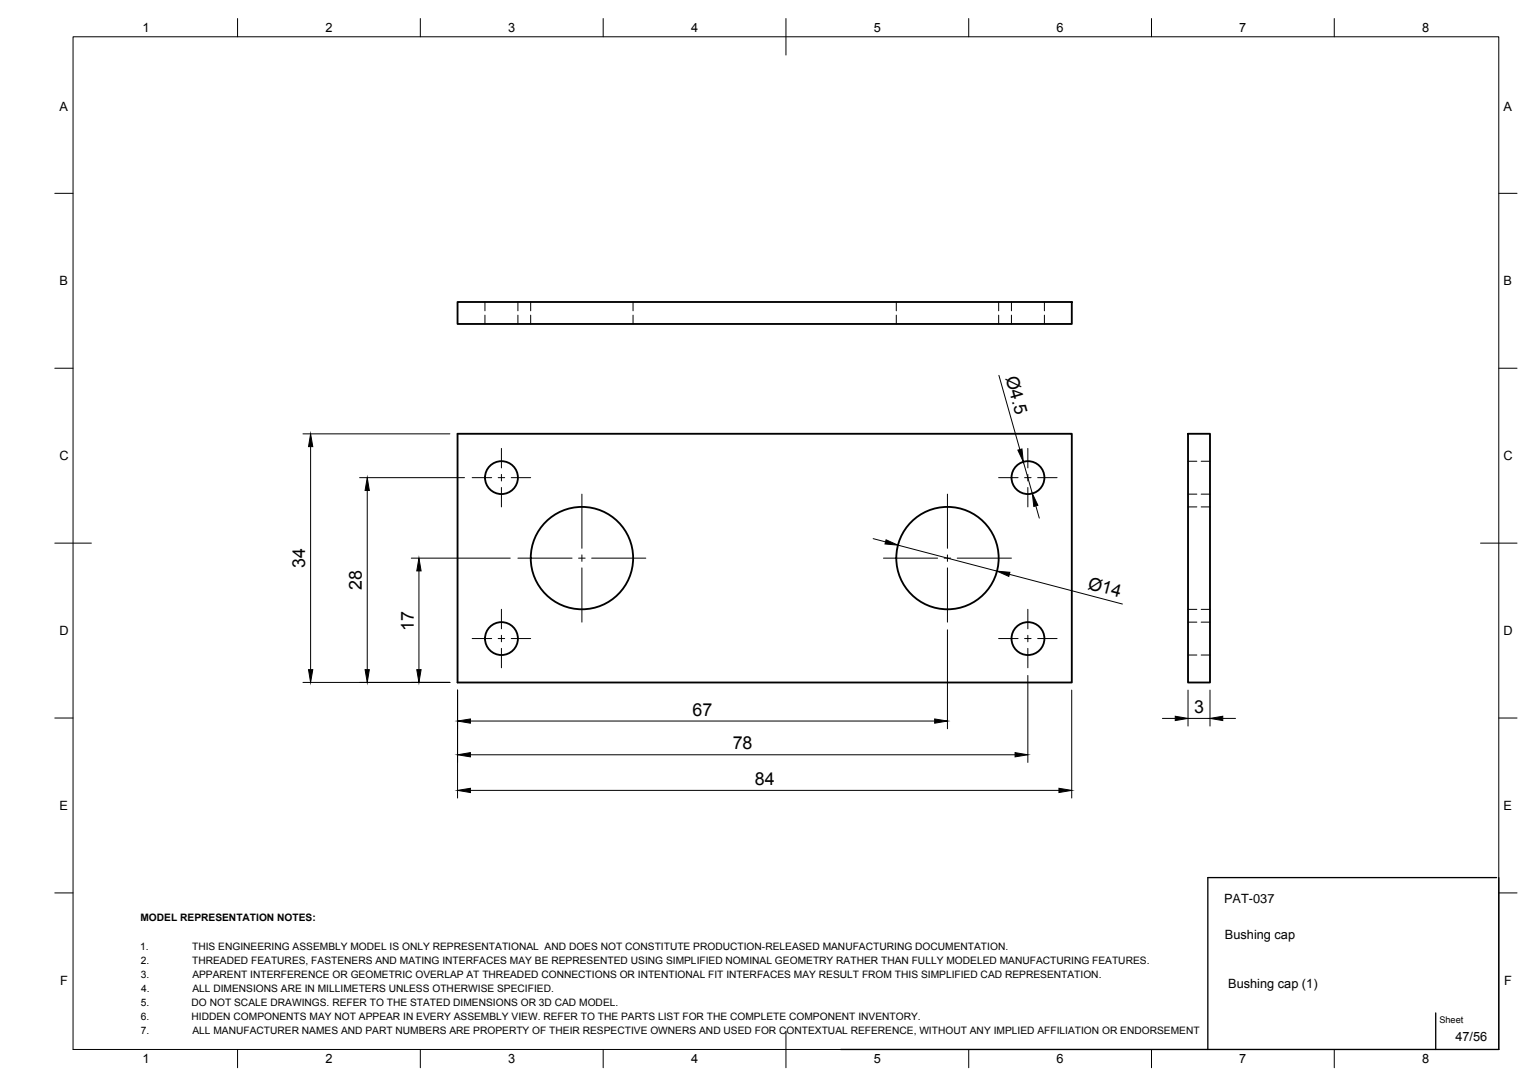
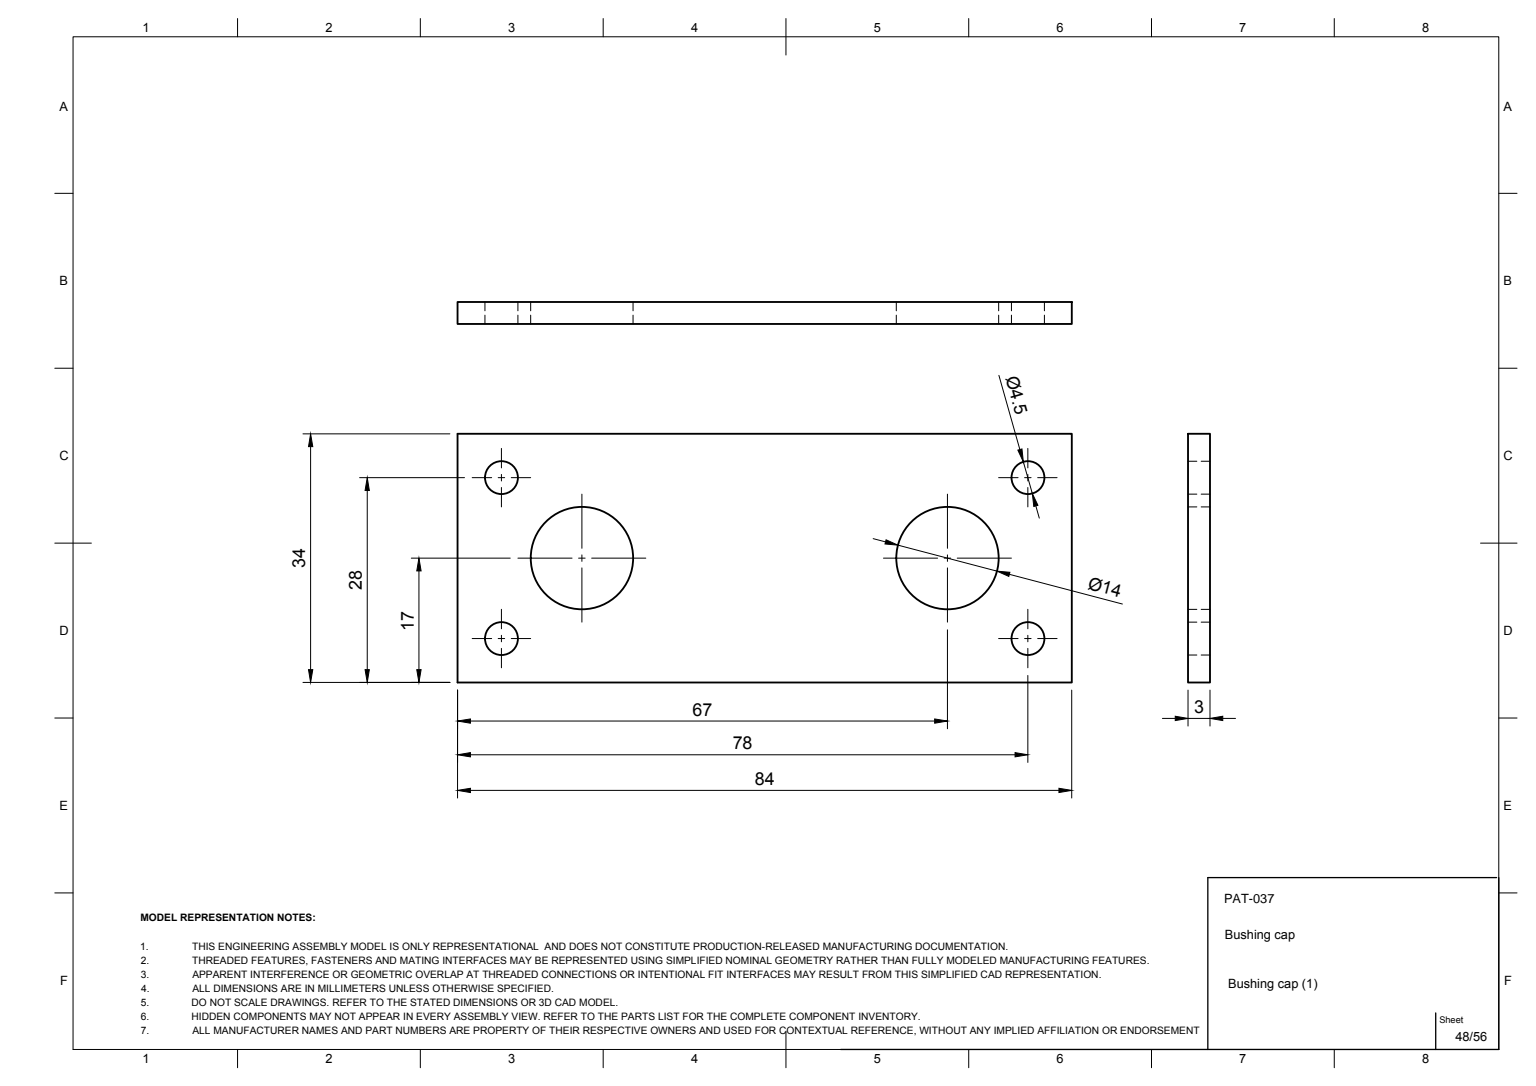
ISO-10303-21;
HEADER;
/* Generated by software containing ST-Developer
 * from STEP Tools, Inc. (www.steptools.com) 
 */

FILE_DESCRIPTION(
/* description */ ('Flywheel Crank-Slider'),
/* implementation_level */ '2;1');

FILE_NAME(
/* name */ 'Bushing cap (1).step',
/* time_stamp */ '2026-10-28T03:23:13-07:00',
/* author */ (''),
/* organization */ (''),
/* preprocessor_version */ 'ST-DEVELOPER v20.2',
/* originating_system */ 'Autodesk Translation Framework v15.17.0.0',
/* authorisation */ '');

FILE_SCHEMA (('AUTOMOTIVE_DESIGN { 1 0 10303 214 3 1 1 }'));
ENDSEC;

DATA;
#10=MECHANICAL_DESIGN_GEOMETRIC_PRESENTATION_REPRESENTATION('',(#721),#17322);
#608=SHAPE_REPRESENTATION_RELATIONSHIP('SRR','None',#17609,#660);
#660=ADVANCED_BREP_SHAPE_REPRESENTATION('',(#778),#17313);
#721=STYLED_ITEM('',(#17924),#778);
#778=MANIFOLD_SOLID_BREP('Body1',#9103);
#979=FACE_BOUND('',#2520,.T.);
#980=FACE_BOUND('',#2521,.T.);
#981=FACE_BOUND('',#2522,.T.);
#982=FACE_BOUND('',#2523,.T.);
#983=FACE_BOUND('',#2524,.T.);
#984=FACE_BOUND('',#2525,.T.);
#985=FACE_BOUND('',#2528,.T.);
#986=FACE_BOUND('',#2529,.T.);
#987=FACE_BOUND('',#2530,.T.);
#988=FACE_BOUND('',#2531,.T.);
#989=FACE_BOUND('',#2532,.T.);
#990=FACE_BOUND('',#2533,.T.);
#1276=PLANE('',#10612);
#1277=PLANE('',#10613);
#1278=PLANE('',#10614);
#1279=PLANE('',#10615);
#1280=PLANE('',#10616);
#1281=PLANE('',#10617);
#1783=FACE_OUTER_BOUND('',#2512,.T.);
#1784=FACE_OUTER_BOUND('',#2513,.T.);
#1785=FACE_OUTER_BOUND('',#2514,.T.);
#1786=FACE_OUTER_BOUND('',#2515,.T.);
#1787=FACE_OUTER_BOUND('',#2516,.T.);
#1788=FACE_OUTER_BOUND('',#2517,.T.);
#1789=FACE_OUTER_BOUND('',#2518,.T.);
#1790=FACE_OUTER_BOUND('',#2519,.T.);
#1791=FACE_OUTER_BOUND('',#2526,.T.);
#1792=FACE_OUTER_BOUND('',#2527,.T.);
#1793=FACE_OUTER_BOUND('',#2534,.T.);
#1794=FACE_OUTER_BOUND('',#2535,.T.);
#2512=EDGE_LOOP('',(#8060,#8061,#8062,#8063));
#2513=EDGE_LOOP('',(#8064,#8065,#8066,#8067));
#2514=EDGE_LOOP('',(#8068,#8069,#8070,#8071));
#2515=EDGE_LOOP('',(#8072,#8073,#8074,#8075));
#2516=EDGE_LOOP('',(#8076,#8077,#8078,#8079));
#2517=EDGE_LOOP('',(#8080,#8081,#8082,#8083));
#2518=EDGE_LOOP('',(#8084,#8085,#8086,#8087));
#2519=EDGE_LOOP('',(#8088,#8089,#8090,#8091));
#2520=EDGE_LOOP('',(#8092));
#2521=EDGE_LOOP('',(#8093));
#2522=EDGE_LOOP('',(#8094));
#2523=EDGE_LOOP('',(#8095));
#2524=EDGE_LOOP('',(#8096));
#2525=EDGE_LOOP('',(#8097));
#2526=EDGE_LOOP('',(#8098,#8099,#8100,#8101));
#2527=EDGE_LOOP('',(#8102,#8103,#8104,#8105));
#2528=EDGE_LOOP('',(#8106));
#2529=EDGE_LOOP('',(#8107));
#2530=EDGE_LOOP('',(#8108));
#2531=EDGE_LOOP('',(#8109));
#2532=EDGE_LOOP('',(#8110));
#2533=EDGE_LOOP('',(#8111));
#2534=EDGE_LOOP('',(#8112,#8113,#8114,#8115));
#2535=EDGE_LOOP('',(#8116,#8117,#8118,#8119));
#3151=LINE('',#16804,#3762);
#3152=LINE('',#16810,#3763);
#3153=LINE('',#16816,#3764);
#3154=LINE('',#16822,#3765);
#3155=LINE('',#16828,#3766);
#3156=LINE('',#16834,#3767);
#3157=LINE('',#16839,#3768);
#3158=LINE('',#16841,#3769);
#3159=LINE('',#16843,#3770);
#3160=LINE('',#16844,#3771);
#3161=LINE('',#16847,#3772);
#3162=LINE('',#16849,#3773);
#3163=LINE('',#16850,#3774);
#3164=LINE('',#16853,#3775);
#3165=LINE('',#16855,#3776);
#3166=LINE('',#16856,#3777);
#3167=LINE('',#16858,#3778);
#3168=LINE('',#16859,#3779);
#3762=VECTOR('',#13187,0.225);
#3763=VECTOR('',#13194,0.225);
#3764=VECTOR('',#13201,0.225);
#3765=VECTOR('',#13208,0.225);
#3766=VECTOR('',#13215,0.7);
#3767=VECTOR('',#13222,0.7);
#3768=VECTOR('',#13227,1.);
#3769=VECTOR('',#13228,1.);
#3770=VECTOR('',#13229,1.);
#3771=VECTOR('',#13230,1.);
#3772=VECTOR('',#13233,1.);
#3773=VECTOR('',#13234,1.);
#3774=VECTOR('',#13235,1.);
#3775=VECTOR('',#13238,1.);
#3776=VECTOR('',#13239,1.);
#3777=VECTOR('',#13240,1.);
#3778=VECTOR('',#13243,1.);
#3779=VECTOR('',#13244,1.);
#4218=CIRCLE('',#10595,0.225);
#4219=CIRCLE('',#10596,0.225);
#4220=CIRCLE('',#10598,0.225);
#4221=CIRCLE('',#10599,0.225);
#4222=CIRCLE('',#10601,0.225);
#4223=CIRCLE('',#10602,0.225);
#4224=CIRCLE('',#10604,0.225);
#4225=CIRCLE('',#10605,0.225);
#4226=CIRCLE('',#10607,0.7);
#4227=CIRCLE('',#10608,0.7);
#4228=CIRCLE('',#10610,0.7);
#4229=CIRCLE('',#10611,0.7);
#4929=VERTEX_POINT('',#16801);
#4930=VERTEX_POINT('',#16803);
#4931=VERTEX_POINT('',#16807);
#4932=VERTEX_POINT('',#16809);
#4933=VERTEX_POINT('',#16813);
#4934=VERTEX_POINT('',#16815);
#4935=VERTEX_POINT('',#16819);
#4936=VERTEX_POINT('',#16821);
#4937=VERTEX_POINT('',#16825);
#4938=VERTEX_POINT('',#16827);
#4939=VERTEX_POINT('',#16831);
#4940=VERTEX_POINT('',#16833);
#4941=VERTEX_POINT('',#16837);
#4942=VERTEX_POINT('',#16838);
#4943=VERTEX_POINT('',#16840);
#4944=VERTEX_POINT('',#16842);
#4945=VERTEX_POINT('',#16846);
#4946=VERTEX_POINT('',#16848);
#4947=VERTEX_POINT('',#16852);
#4948=VERTEX_POINT('',#16854);
#5987=EDGE_CURVE('',#4929,#4929,#4218,.T.);
#5988=EDGE_CURVE('',#4929,#4930,#3151,.T.);
#5989=EDGE_CURVE('',#4930,#4930,#4219,.T.);
#5990=EDGE_CURVE('',#4931,#4931,#4220,.T.);
#5991=EDGE_CURVE('',#4931,#4932,#3152,.T.);
#5992=EDGE_CURVE('',#4932,#4932,#4221,.T.);
#5993=EDGE_CURVE('',#4933,#4933,#4222,.T.);
#5994=EDGE_CURVE('',#4933,#4934,#3153,.T.);
#5995=EDGE_CURVE('',#4934,#4934,#4223,.T.);
#5996=EDGE_CURVE('',#4935,#4935,#4224,.T.);
#5997=EDGE_CURVE('',#4935,#4936,#3154,.T.);
#5998=EDGE_CURVE('',#4936,#4936,#4225,.T.);
#5999=EDGE_CURVE('',#4937,#4937,#4226,.T.);
#6000=EDGE_CURVE('',#4937,#4938,#3155,.T.);
#6001=EDGE_CURVE('',#4938,#4938,#4227,.T.);
#6002=EDGE_CURVE('',#4939,#4939,#4228,.T.);
#6003=EDGE_CURVE('',#4939,#4940,#3156,.T.);
#6004=EDGE_CURVE('',#4940,#4940,#4229,.T.);
#6005=EDGE_CURVE('',#4941,#4942,#3157,.T.);
#6006=EDGE_CURVE('',#4942,#4943,#3158,.T.);
#6007=EDGE_CURVE('',#4944,#4943,#3159,.T.);
#6008=EDGE_CURVE('',#4941,#4944,#3160,.T.);
#6009=EDGE_CURVE('',#4945,#4941,#3161,.T.);
#6010=EDGE_CURVE('',#4946,#4944,#3162,.T.);
#6011=EDGE_CURVE('',#4945,#4946,#3163,.T.);
#6012=EDGE_CURVE('',#4947,#4945,#3164,.T.);
#6013=EDGE_CURVE('',#4948,#4946,#3165,.T.);
#6014=EDGE_CURVE('',#4947,#4948,#3166,.T.);
#6015=EDGE_CURVE('',#4942,#4947,#3167,.T.);
#6016=EDGE_CURVE('',#4943,#4948,#3168,.T.);
#8060=ORIENTED_EDGE('',*,*,#5987,.F.);
#8061=ORIENTED_EDGE('',*,*,#5988,.T.);
#8062=ORIENTED_EDGE('',*,*,#5989,.F.);
#8063=ORIENTED_EDGE('',*,*,#5988,.F.);
#8064=ORIENTED_EDGE('',*,*,#5990,.F.);
#8065=ORIENTED_EDGE('',*,*,#5991,.T.);
#8066=ORIENTED_EDGE('',*,*,#5992,.F.);
#8067=ORIENTED_EDGE('',*,*,#5991,.F.);
#8068=ORIENTED_EDGE('',*,*,#5993,.F.);
#8069=ORIENTED_EDGE('',*,*,#5994,.T.);
#8070=ORIENTED_EDGE('',*,*,#5995,.F.);
#8071=ORIENTED_EDGE('',*,*,#5994,.F.);
#8072=ORIENTED_EDGE('',*,*,#5996,.F.);
#8073=ORIENTED_EDGE('',*,*,#5997,.T.);
#8074=ORIENTED_EDGE('',*,*,#5998,.F.);
#8075=ORIENTED_EDGE('',*,*,#5997,.F.);
#8076=ORIENTED_EDGE('',*,*,#5999,.F.);
#8077=ORIENTED_EDGE('',*,*,#6000,.T.);
#8078=ORIENTED_EDGE('',*,*,#6001,.F.);
#8079=ORIENTED_EDGE('',*,*,#6000,.F.);
#8080=ORIENTED_EDGE('',*,*,#6002,.F.);
#8081=ORIENTED_EDGE('',*,*,#6003,.T.);
#8082=ORIENTED_EDGE('',*,*,#6004,.F.);
#8083=ORIENTED_EDGE('',*,*,#6003,.F.);
#8084=ORIENTED_EDGE('',*,*,#6005,.T.);
#8085=ORIENTED_EDGE('',*,*,#6006,.T.);
#8086=ORIENTED_EDGE('',*,*,#6007,.F.);
#8087=ORIENTED_EDGE('',*,*,#6008,.F.);
#8088=ORIENTED_EDGE('',*,*,#6009,.T.);
#8089=ORIENTED_EDGE('',*,*,#6008,.T.);
#8090=ORIENTED_EDGE('',*,*,#6010,.F.);
#8091=ORIENTED_EDGE('',*,*,#6011,.F.);
#8092=ORIENTED_EDGE('',*,*,#6004,.T.);
#8093=ORIENTED_EDGE('',*,*,#6001,.T.);
#8094=ORIENTED_EDGE('',*,*,#5998,.T.);
#8095=ORIENTED_EDGE('',*,*,#5995,.T.);
#8096=ORIENTED_EDGE('',*,*,#5992,.T.);
#8097=ORIENTED_EDGE('',*,*,#5989,.T.);
#8098=ORIENTED_EDGE('',*,*,#6012,.T.);
#8099=ORIENTED_EDGE('',*,*,#6011,.T.);
#8100=ORIENTED_EDGE('',*,*,#6013,.F.);
#8101=ORIENTED_EDGE('',*,*,#6014,.F.);
#8102=ORIENTED_EDGE('',*,*,#6015,.T.);
#8103=ORIENTED_EDGE('',*,*,#6014,.T.);
#8104=ORIENTED_EDGE('',*,*,#6016,.F.);
#8105=ORIENTED_EDGE('',*,*,#6006,.F.);
#8106=ORIENTED_EDGE('',*,*,#6002,.T.);
#8107=ORIENTED_EDGE('',*,*,#5999,.T.);
#8108=ORIENTED_EDGE('',*,*,#5996,.T.);
#8109=ORIENTED_EDGE('',*,*,#5993,.T.);
#8110=ORIENTED_EDGE('',*,*,#5990,.T.);
#8111=ORIENTED_EDGE('',*,*,#5987,.T.);
#8112=ORIENTED_EDGE('',*,*,#6016,.T.);
#8113=ORIENTED_EDGE('',*,*,#6013,.T.);
#8114=ORIENTED_EDGE('',*,*,#6010,.T.);
#8115=ORIENTED_EDGE('',*,*,#6007,.T.);
#8116=ORIENTED_EDGE('',*,*,#6015,.F.);
#8117=ORIENTED_EDGE('',*,*,#6005,.F.);
#8118=ORIENTED_EDGE('',*,*,#6009,.F.);
#8119=ORIENTED_EDGE('',*,*,#6012,.F.);
#8486=CYLINDRICAL_SURFACE('',#10594,0.225);
#8487=CYLINDRICAL_SURFACE('',#10597,0.225);
#8488=CYLINDRICAL_SURFACE('',#10600,0.225);
#8489=CYLINDRICAL_SURFACE('',#10603,0.225);
#8490=CYLINDRICAL_SURFACE('',#10606,0.7);
#8491=CYLINDRICAL_SURFACE('',#10609,0.7);
#8974=ADVANCED_FACE('',(#1783),#8486,.F.);
#8975=ADVANCED_FACE('',(#1784),#8487,.F.);
#8976=ADVANCED_FACE('',(#1785),#8488,.F.);
#8977=ADVANCED_FACE('',(#1786),#8489,.F.);
#8978=ADVANCED_FACE('',(#1787),#8490,.F.);
#8979=ADVANCED_FACE('',(#1788),#8491,.F.);
#8980=ADVANCED_FACE('',(#1789),#1276,.T.);
#8981=ADVANCED_FACE('',(#1790,#979,#980,#981,#982,#983,#984),#1277,.T.);
#8982=ADVANCED_FACE('',(#1791),#1278,.T.);
#8983=ADVANCED_FACE('',(#1792,#985,#986,#987,#988,#989,#990),#1279,.T.);
#8984=ADVANCED_FACE('',(#1793),#1280,.T.);
#8985=ADVANCED_FACE('',(#1794),#1281,.F.);
#9103=CLOSED_SHELL('',(#8974,#8975,#8976,#8977,#8978,#8979,#8980,#8981,
#8982,#8983,#8984,#8985));
#10593=AXIS2_PLACEMENT_3D('',#16799,#13181,#13182);
#10594=AXIS2_PLACEMENT_3D('',#16800,#13183,#13184);
#10595=AXIS2_PLACEMENT_3D('',#16802,#13185,#13186);
#10596=AXIS2_PLACEMENT_3D('',#16805,#13188,#13189);
#10597=AXIS2_PLACEMENT_3D('',#16806,#13190,#13191);
#10598=AXIS2_PLACEMENT_3D('',#16808,#13192,#13193);
#10599=AXIS2_PLACEMENT_3D('',#16811,#13195,#13196);
#10600=AXIS2_PLACEMENT_3D('',#16812,#13197,#13198);
#10601=AXIS2_PLACEMENT_3D('',#16814,#13199,#13200);
#10602=AXIS2_PLACEMENT_3D('',#16817,#13202,#13203);
#10603=AXIS2_PLACEMENT_3D('',#16818,#13204,#13205);
#10604=AXIS2_PLACEMENT_3D('',#16820,#13206,#13207);
#10605=AXIS2_PLACEMENT_3D('',#16823,#13209,#13210);
#10606=AXIS2_PLACEMENT_3D('',#16824,#13211,#13212);
#10607=AXIS2_PLACEMENT_3D('',#16826,#13213,#13214);
#10608=AXIS2_PLACEMENT_3D('',#16829,#13216,#13217);
#10609=AXIS2_PLACEMENT_3D('',#16830,#13218,#13219);
#10610=AXIS2_PLACEMENT_3D('',#16832,#13220,#13221);
#10611=AXIS2_PLACEMENT_3D('',#16835,#13223,#13224);
#10612=AXIS2_PLACEMENT_3D('',#16836,#13225,#13226);
#10613=AXIS2_PLACEMENT_3D('',#16845,#13231,#13232);
#10614=AXIS2_PLACEMENT_3D('',#16851,#13236,#13237);
#10615=AXIS2_PLACEMENT_3D('',#16857,#13241,#13242);
#10616=AXIS2_PLACEMENT_3D('',#16860,#13245,#13246);
#10617=AXIS2_PLACEMENT_3D('',#16861,#13247,#13248);
#13181=DIRECTION('axis',(0.,0.,1.));
#13182=DIRECTION('refdir',(1.,0.,0.));
#13183=DIRECTION('center_axis',(1.,0.,0.));
#13184=DIRECTION('ref_axis',(0.,0.,-1.));
#13185=DIRECTION('center_axis',(1.,0.,0.));
#13186=DIRECTION('ref_axis',(0.,0.,-1.));
#13187=DIRECTION('',(1.,0.,0.));
#13188=DIRECTION('center_axis',(-1.,0.,0.));
#13189=DIRECTION('ref_axis',(0.,0.,-1.));
#13190=DIRECTION('center_axis',(1.,0.,0.));
#13191=DIRECTION('ref_axis',(0.,0.,-1.));
#13192=DIRECTION('center_axis',(1.,0.,0.));
#13193=DIRECTION('ref_axis',(0.,0.,-1.));
#13194=DIRECTION('',(1.,0.,0.));
#13195=DIRECTION('center_axis',(-1.,0.,0.));
#13196=DIRECTION('ref_axis',(0.,0.,-1.));
#13197=DIRECTION('center_axis',(1.,0.,0.));
#13198=DIRECTION('ref_axis',(0.,0.,-1.));
#13199=DIRECTION('center_axis',(1.,0.,0.));
#13200=DIRECTION('ref_axis',(0.,0.,-1.));
#13201=DIRECTION('',(1.,0.,0.));
#13202=DIRECTION('center_axis',(-1.,0.,0.));
#13203=DIRECTION('ref_axis',(0.,0.,-1.));
#13204=DIRECTION('center_axis',(1.,0.,0.));
#13205=DIRECTION('ref_axis',(0.,0.,-1.));
#13206=DIRECTION('center_axis',(1.,0.,0.));
#13207=DIRECTION('ref_axis',(0.,0.,-1.));
#13208=DIRECTION('',(1.,0.,0.));
#13209=DIRECTION('center_axis',(-1.,0.,0.));
#13210=DIRECTION('ref_axis',(0.,0.,-1.));
#13211=DIRECTION('center_axis',(1.,0.,0.));
#13212=DIRECTION('ref_axis',(0.,0.,-1.));
#13213=DIRECTION('center_axis',(1.,0.,0.));
#13214=DIRECTION('ref_axis',(0.,0.,-1.));
#13215=DIRECTION('',(1.,0.,0.));
#13216=DIRECTION('center_axis',(-1.,0.,0.));
#13217=DIRECTION('ref_axis',(0.,0.,-1.));
#13218=DIRECTION('center_axis',(1.,0.,0.));
#13219=DIRECTION('ref_axis',(0.,0.,-1.));
#13220=DIRECTION('center_axis',(1.,0.,0.));
#13221=DIRECTION('ref_axis',(0.,0.,-1.));
#13222=DIRECTION('',(1.,0.,0.));
#13223=DIRECTION('center_axis',(-1.,0.,0.));
#13224=DIRECTION('ref_axis',(0.,0.,-1.));
#13225=DIRECTION('center_axis',(0.,1.,0.));
#13226=DIRECTION('ref_axis',(-1.,0.,0.));
#13227=DIRECTION('',(-1.,0.,0.));
#13228=DIRECTION('',(0.,0.,1.));
#13229=DIRECTION('',(-1.,0.,0.));
#13230=DIRECTION('',(0.,0.,1.));
#13231=DIRECTION('center_axis',(1.,0.,0.));
#13232=DIRECTION('ref_axis',(0.,1.,0.));
#13233=DIRECTION('',(0.,1.,0.));
#13234=DIRECTION('',(0.,1.,0.));
#13235=DIRECTION('',(0.,0.,1.));
#13236=DIRECTION('center_axis',(0.,-1.,0.));
#13237=DIRECTION('ref_axis',(1.,0.,0.));
#13238=DIRECTION('',(1.,0.,0.));
#13239=DIRECTION('',(1.,0.,0.));
#13240=DIRECTION('',(0.,0.,1.));
#13241=DIRECTION('center_axis',(-1.,0.,0.));
#13242=DIRECTION('ref_axis',(0.,-1.,0.));
#13243=DIRECTION('',(0.,-1.,0.));
#13244=DIRECTION('',(0.,-1.,0.));
#13245=DIRECTION('center_axis',(0.,0.,1.));
#13246=DIRECTION('ref_axis',(1.,0.,0.));
#13247=DIRECTION('center_axis',(0.,0.,1.));
#13248=DIRECTION('ref_axis',(1.,0.,0.));
#16799=CARTESIAN_POINT('',(0.,0.,0.));
#16800=CARTESIAN_POINT('Origin',(13.5,3.6,3.9));
#16801=CARTESIAN_POINT('',(13.6,3.6,4.125));
#16802=CARTESIAN_POINT('Origin',(13.6,3.6,3.9));
#16803=CARTESIAN_POINT('',(13.9,3.6,4.125));
#16804=CARTESIAN_POINT('',(13.5,3.6,4.125));
#16805=CARTESIAN_POINT('Origin',(13.9,3.6,3.9));
#16806=CARTESIAN_POINT('Origin',(13.5,-3.6,6.1));
#16807=CARTESIAN_POINT('',(13.6,-3.6,6.325));
#16808=CARTESIAN_POINT('Origin',(13.6,-3.6,6.1));
#16809=CARTESIAN_POINT('',(13.9,-3.6,6.325));
#16810=CARTESIAN_POINT('',(13.5,-3.6,6.325));
#16811=CARTESIAN_POINT('Origin',(13.9,-3.6,6.1));
#16812=CARTESIAN_POINT('Origin',(13.5,-3.6,3.9));
#16813=CARTESIAN_POINT('',(13.6,-3.6,4.125));
#16814=CARTESIAN_POINT('Origin',(13.6,-3.6,3.9));
#16815=CARTESIAN_POINT('',(13.9,-3.6,4.125));
#16816=CARTESIAN_POINT('',(13.5,-3.6,4.125));
#16817=CARTESIAN_POINT('Origin',(13.9,-3.6,3.9));
#16818=CARTESIAN_POINT('Origin',(13.5,3.6,6.1));
#16819=CARTESIAN_POINT('',(13.6,3.6,6.325));
#16820=CARTESIAN_POINT('Origin',(13.6,3.6,6.1));
#16821=CARTESIAN_POINT('',(13.9,3.6,6.325));
#16822=CARTESIAN_POINT('',(13.5,3.6,6.325));
#16823=CARTESIAN_POINT('Origin',(13.9,3.6,6.1));
#16824=CARTESIAN_POINT('Origin',(13.5,-2.5,5.));
#16825=CARTESIAN_POINT('',(13.6,-2.5,5.7));
#16826=CARTESIAN_POINT('Origin',(13.6,-2.5,5.));
#16827=CARTESIAN_POINT('',(13.9,-2.5,5.7));
#16828=CARTESIAN_POINT('',(13.5,-2.5,5.7));
#16829=CARTESIAN_POINT('Origin',(13.9,-2.5,5.));
#16830=CARTESIAN_POINT('Origin',(13.5,2.5,5.));
#16831=CARTESIAN_POINT('',(13.6,2.5,5.7));
#16832=CARTESIAN_POINT('Origin',(13.6,2.5,5.));
#16833=CARTESIAN_POINT('',(13.9,2.5,5.7));
#16834=CARTESIAN_POINT('',(13.5,2.5,5.7));
#16835=CARTESIAN_POINT('Origin',(13.9,2.5,5.));
#16836=CARTESIAN_POINT('Origin',(13.9,4.2,3.3));
#16837=CARTESIAN_POINT('',(13.9,4.2,3.3));
#16838=CARTESIAN_POINT('',(13.6,4.2,3.3));
#16839=CARTESIAN_POINT('',(13.9,4.2,3.3));
#16840=CARTESIAN_POINT('',(13.6,4.2,6.7));
#16841=CARTESIAN_POINT('',(13.6,4.2,3.3));
#16842=CARTESIAN_POINT('',(13.9,4.2,6.7));
#16843=CARTESIAN_POINT('',(13.9,4.2,6.7));
#16844=CARTESIAN_POINT('',(13.9,4.2,3.3));
#16845=CARTESIAN_POINT('Origin',(13.9,-4.2,3.3));
#16846=CARTESIAN_POINT('',(13.9,-4.2,3.3));
#16847=CARTESIAN_POINT('',(13.9,-4.2,3.3));
#16848=CARTESIAN_POINT('',(13.9,-4.2,6.7));
#16849=CARTESIAN_POINT('',(13.9,-4.2,6.7));
#16850=CARTESIAN_POINT('',(13.9,-4.2,3.3));
#16851=CARTESIAN_POINT('Origin',(13.6,-4.2,3.3));
#16852=CARTESIAN_POINT('',(13.6,-4.2,3.3));
#16853=CARTESIAN_POINT('',(13.6,-4.2,3.3));
#16854=CARTESIAN_POINT('',(13.6,-4.2,6.7));
#16855=CARTESIAN_POINT('',(13.6,-4.2,6.7));
#16856=CARTESIAN_POINT('',(13.6,-4.2,3.3));
#16857=CARTESIAN_POINT('Origin',(13.6,4.2,3.3));
#16858=CARTESIAN_POINT('',(13.6,4.2,3.3));
#16859=CARTESIAN_POINT('',(13.6,4.2,6.7));
#16860=CARTESIAN_POINT('Origin',(13.75,0.,6.7));
#16861=CARTESIAN_POINT('Origin',(13.75,0.,3.3));
#17252=UNCERTAINTY_MEASURE_WITH_UNIT(LENGTH_MEASURE(0.001),#17323,
'DISTANCE_ACCURACY_VALUE',
'Maximum model space distance between geometric entities at asserted c
onnectivities');
#17261=UNCERTAINTY_MEASURE_WITH_UNIT(LENGTH_MEASURE(0.001),#17323,
'DISTANCE_ACCURACY_VALUE',
'Maximum model space distance between geometric entities at asserted c
onnectivities');
#17313=(
GEOMETRIC_REPRESENTATION_CONTEXT(3)
GLOBAL_UNCERTAINTY_ASSIGNED_CONTEXT((#17252))
GLOBAL_UNIT_ASSIGNED_CONTEXT((#17323,#17325,#17326))
REPRESENTATION_CONTEXT('','3D')
);
#17322=(
GEOMETRIC_REPRESENTATION_CONTEXT(3)
GLOBAL_UNCERTAINTY_ASSIGNED_CONTEXT((#17261))
GLOBAL_UNIT_ASSIGNED_CONTEXT((#17323,#17325,#17326))
REPRESENTATION_CONTEXT('','3D')
);
#17323=(
LENGTH_UNIT()
NAMED_UNIT(*)
SI_UNIT(.CENTI.,.METRE.)
);
#17325=(
NAMED_UNIT(*)
PLANE_ANGLE_UNIT()
SI_UNIT($,.RADIAN.)
);
#17326=(
NAMED_UNIT(*)
SI_UNIT($,.STERADIAN.)
SOLID_ANGLE_UNIT()
);
#17378=SHAPE_DEFINITION_REPRESENTATION(#17452,#17609);
#17452=PRODUCT_DEFINITION_SHAPE('',$,#17670);
#17609=SHAPE_REPRESENTATION('',(#10593),#17313);
#17618=PRODUCT_DEFINITION_CONTEXT('part definition',#17800,'design');
#17670=PRODUCT_DEFINITION('Bushing cap (1)','Bushing cap (1)',#17730,#17618);
#17730=PRODUCT_DEFINITION_FORMATION('',$,#17853);
#17800=APPLICATION_CONTEXT(
'Core Data for Automotive Mechanical Design Process');
#17801=PRODUCT_CONTEXT('part definition',#17800,'mechanical');
#17853=PRODUCT('Bushing cap (1)','Bushing cap (1)','Bushing cap (1)',(#17801));
#17918=COLOUR_RGB('Sky Blue',0.24,0.69,0.87);
#17919=FILL_AREA_STYLE_COLOUR('',#17918);
#17920=FILL_AREA_STYLE('',(#17919));
#17921=SURFACE_STYLE_FILL_AREA(#17920);
#17922=SURFACE_SIDE_STYLE('',(#17921));
#17923=SURFACE_STYLE_USAGE(.BOTH.,#17922);
#17924=PRESENTATION_STYLE_ASSIGNMENT((#17923));
ENDSEC;
END-ISO-10303-21;
